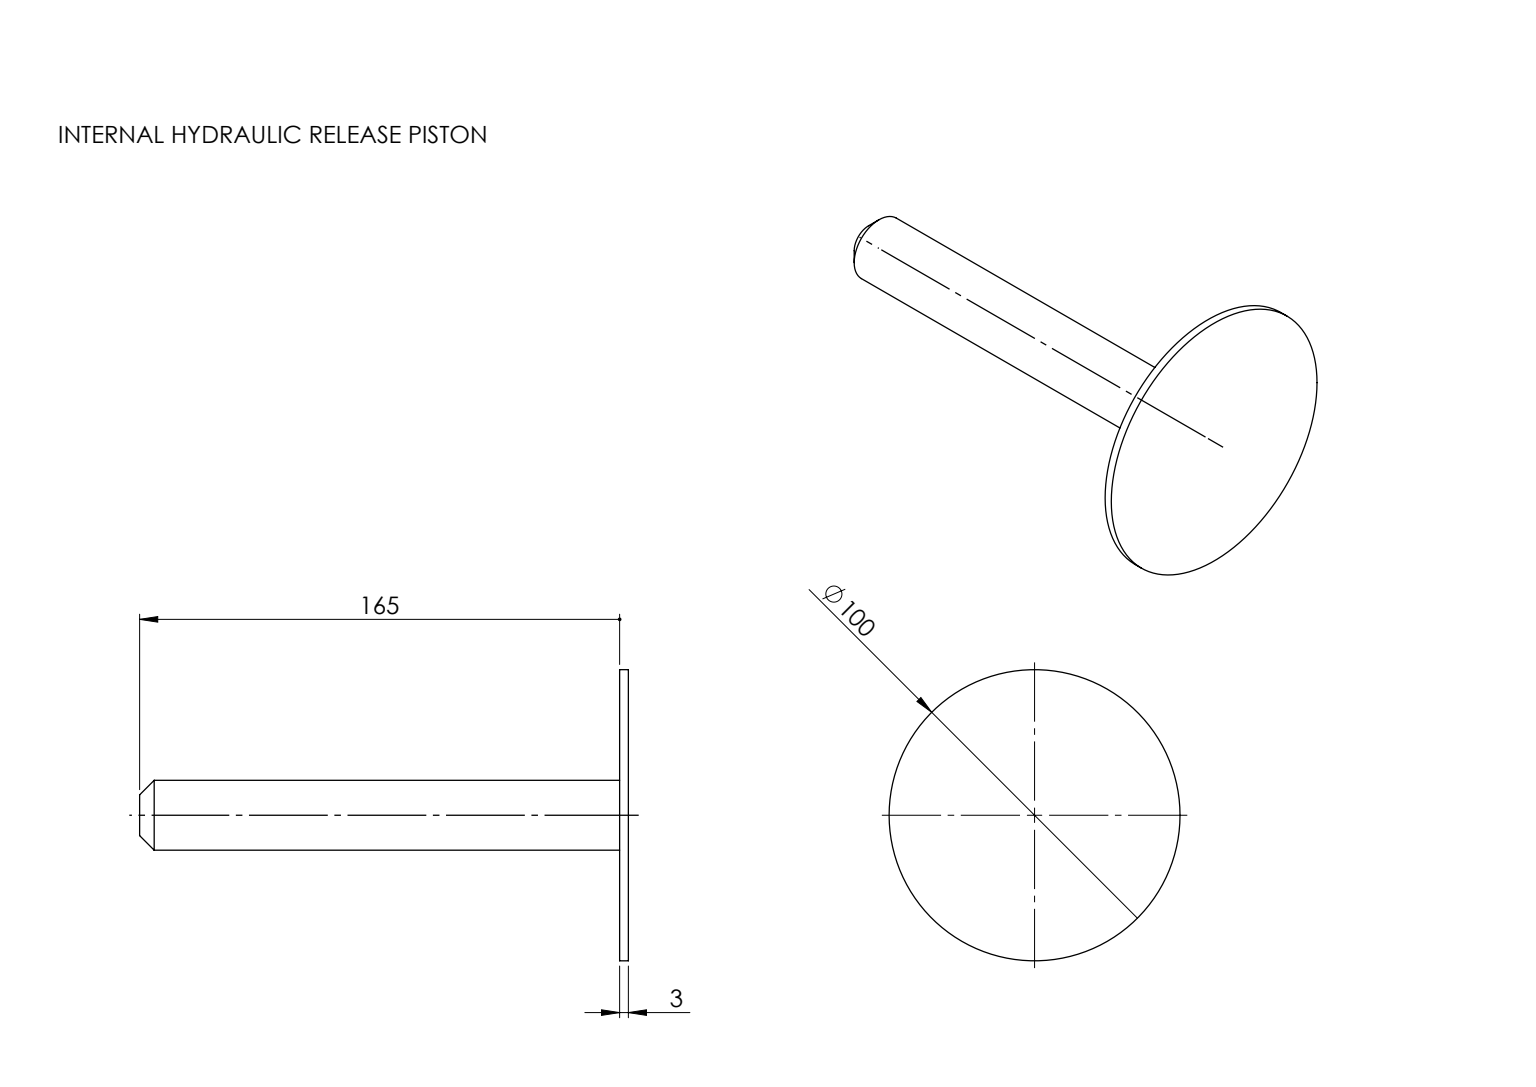
ISO-10303-21;
HEADER;
FILE_DESCRIPTION (('STEP AP214'),
    '1' );
FILE_NAME ('Internal Hydraulic Release Piston.step',
    '2026-10-08T07:58:12',
    ( '' ),
    ( '' ),
    'SwSTEP 2.0',
    'SolidWorks 2026',
    '' );
FILE_SCHEMA (( 'AUTOMOTIVE_DESIGN' ));
ENDSEC;

DATA;
#3=CARTESIAN_POINT ( 'NONE',  ( 112.4999999999999858, 155.0000000000000000, -6.938893903907228378E-15 ) ) ;
#34=EDGE_LOOP ( 'NONE', ( #21556, #29225, #7331, #33094 ) ) ;
#120=ORIENTED_EDGE ( 'NONE', *, *, #31535, .T. ) ;
#168=FILL_AREA_STYLE ('',( #5443 ) ) ;
#368=VECTOR ( 'NONE', #30488, 1000.000000000000000 ) ;
#375=MECHANICAL_DESIGN_GEOMETRIC_PRESENTATION_REPRESENTATION('',(#3643),#27015);
#385=DIRECTION ( 'NONE',  ( -1.000000000000000000, -0.000000000000000000, -0.000000000000000000 ) ) ;
#394=VECTOR ( 'NONE', #33049, 1000.000000000000114 ) ;
#409=EDGE_LOOP ( 'NONE', ( #12808, #6354, #120, #4248 ) ) ;
#672=MANIFOLD_SOLID_BREP ( 'Boss-Extrude2', #22647 ) ;
#768=ORIENTED_EDGE ( 'NONE', *, *, #31535, .F. ) ;
#874=DIRECTION ( 'NONE',  ( 1.000000000000000000, 0.000000000000000000, 0.000000000000000000 ) ) ;
#999=DIRECTION ( 'NONE',  ( 0.000000000000000000, 0.000000000000000000, 1.000000000000000000 ) ) ;
#1205=PRESENTATION_STYLE_ASSIGNMENT (( #14154 ) ) ;
#1257=PRODUCT ( 'Internal Hydraulic Release Piston', 'Internal Hydraulic Release Piston', '', ( #26899 ) ) ;
#1290=AXIS2_PLACEMENT_3D ( 'NONE', #17289, #33134, #30578 ) ;
#1337=VERTEX_POINT ( 'NONE', #24281 ) ;
#1508=AXIS2_PLACEMENT_3D ( 'NONE', #25293, #33136, #15242 ) ;
#1607=EDGE_CURVE ( 'NONE', #8578, #22189, #6963, .T. ) ;
#1664=VERTEX_POINT ( 'NONE', #18314 ) ;
#1670=EDGE_CURVE ( 'NONE', #22189, #8578, #14617, .T. ) ;
#1776=EDGE_LOOP ( 'NONE', ( #1876, #22480, #11969, #27098 ) ) ;
#1840=CYLINDRICAL_SURFACE ( 'NONE', #11781, 12.00000000000000355 ) ;
#1876=ORIENTED_EDGE ( 'NONE', *, *, #16847, .F. ) ;
#1924=ORIENTED_EDGE ( 'NONE', *, *, #23365, .F. ) ;
#2147=CARTESIAN_POINT ( 'NONE',  ( 112.4999999999999858, 155.0000000000000000, -6.938893903907228378E-15 ) ) ;
#2185=SHAPE_REPRESENTATION ( 'Internal Hydraulic Release Piston', ( #2404 ), #27952 ) ;
#2223=DIRECTION ( 'NONE',  ( -1.000000000000000000, -0.000000000000000000, -0.000000000000000000 ) ) ;
#2250=DIRECTION ( 'NONE',  ( 0.000000000000000000, 0.000000000000000000, -1.000000000000000000 ) ) ;
#2404=AXIS2_PLACEMENT_3D ( 'NONE', #8872, #11941, #4266 ) ;
#2565=SHAPE_REPRESENTATION_RELATIONSHIP ( 'NONE' , 'NONE' ,  #2185, #14909 ) ;
#2939=COLOUR_RGB ( '', 0.66274510, 0.83137255, 0.94901961) ;
#3015=FACE_OUTER_BOUND ( 'NONE', #1776, .T. ) ;
#3175=DIRECTION ( 'NONE',  ( -1.000000000000000000, -0.000000000000000000, -0.000000000000000000 ) ) ;
#3218=CARTESIAN_POINT ( 'NONE',  ( 115.4999999999999858, 155.0000000000000000, -6.938893903907228378E-15 ) ) ;
#3386=SHAPE_DEFINITION_REPRESENTATION ( #33668, #2185 ) ;
#3476=( GEOMETRIC_REPRESENTATION_CONTEXT ( 3 ) GLOBAL_UNCERTAINTY_ASSIGNED_CONTEXT ( ( #16111 ) ) GLOBAL_UNIT_ASSIGNED_CONTEXT ( ( #32711, #27439, #10407 ) ) REPRESENTATION_CONTEXT ( 'NONE', 'WORKASPACE' ) );
#3643=STYLED_ITEM ( 'NONE', ( #24499 ), #672 ) ;
#3732=DIRECTION ( 'NONE',  ( 1.000000000000000000, 0.000000000000000000, 0.000000000000000000 ) ) ;
#3769=FILL_AREA_STYLE ('',( #27108 ) ) ;
#4018=MECHANICAL_DESIGN_GEOMETRIC_PRESENTATION_REPRESENTATION('',(#13819),#3476);
#4163=EDGE_CURVE ( 'NONE', #8578, #31129, #13331, .T. ) ;
#4176=CARTESIAN_POINT ( 'NONE',  ( 112.4999999999999858, 155.0000000000000000, -6.938893903907228378E-15 ) ) ;
#4218=DIRECTION ( 'NONE',  ( 0.000000000000000000, 0.000000000000000000, 1.000000000000000000 ) ) ;
#4248=ORIENTED_EDGE ( 'NONE', *, *, #25720, .T. ) ;
#4266=DIRECTION ( 'NONE',  ( 1.000000000000000000, 0.000000000000000000, 0.000000000000000000 ) ) ;
#4522=DIRECTION ( 'NONE',  ( 0.000000000000000000, 0.000000000000000000, -1.000000000000000000 ) ) ;
#4904=LINE ( 'NONE', #22961, #7980 ) ;
#5202=EDGE_CURVE ( 'NONE', #1337, #29025, #8726, .T. ) ;
#5443=FILL_AREA_STYLE_COLOUR ( '', #24313 ) ;
#5628=AXIS2_PLACEMENT_3D ( 'NONE', #4176, #19521, #4522 ) ;
#5888=UNCERTAINTY_MEASURE_WITH_UNIT (LENGTH_MEASURE( 1.000000000000000082E-05 ), #26387, 'distance_accuracy_value', 'NONE');
#6054=VECTOR ( 'NONE', #385, 1000.000000000000000 ) ;
#6112=AXIS2_PLACEMENT_3D ( 'NONE', #22939, #14935, #9482 ) ;
#6312=( NAMED_UNIT ( * ) PLANE_ANGLE_UNIT ( ) SI_UNIT ( $, .RADIAN. ) );
#6354=ORIENTED_EDGE ( 'NONE', *, *, #1670, .F. ) ;
#6598=EDGE_LOOP ( 'NONE', ( #10063, #33597, #18191, #768 ) ) ;
#6737=AXIS2_PLACEMENT_3D ( 'NONE', #20804, #7872, #20130 ) ;
#6963=CIRCLE ( 'NONE', #26011, 12.00000000000000355 ) ;
#7331=ORIENTED_EDGE ( 'NONE', *, *, #29781, .T. ) ;
#7508=CIRCLE ( 'NONE', #1508, 50.00000000000000000 ) ;
#7830=LINE ( 'NONE', #33213, #368 ) ;
#7872=DIRECTION ( 'NONE',  ( 1.000000000000000000, -0.000000000000000000, -0.000000000000000000 ) ) ;
#7939=DIRECTION ( 'NONE',  ( 0.000000000000000000, 0.000000000000000000, -1.000000000000000000 ) ) ;
#7980=VECTOR ( 'NONE', #22285, 1000.000000000000000 ) ;
#7987=CARTESIAN_POINT ( 'NONE',  ( 112.4999999999999858, 155.0000000000000000, -50.00000000000000711 ) ) ;
#8143=CARTESIAN_POINT ( 'NONE',  ( -47.49999999999998579, 155.0000000000000000, -6.938893903907228378E-15 ) ) ;
#8320=CIRCLE ( 'NONE', #6112, 6.999999999999950262 ) ;
#8578=VERTEX_POINT ( 'NONE', #16343 ) ;
#8726=CIRCLE ( 'NONE', #9827, 50.00000000000000000 ) ;
#8740=PRODUCT_DEFINITION_CONTEXT ( 'detailed design', #14200, 'design' ) ;
#8872=CARTESIAN_POINT ( 'NONE',  ( 0.000000000000000000, 0.000000000000000000, 0.000000000000000000 ) ) ;
#8976=APPLICATION_CONTEXT ( 'automotive_design' ) ;
#8992=CARTESIAN_POINT ( 'NONE',  ( -47.49999999999998579, 155.0000000000000000, -6.938893903907228378E-15 ) ) ;
#9056=EDGE_LOOP ( 'NONE', ( #32117, #30050 ) ) ;
#9124=FACE_OUTER_BOUND ( 'NONE', #9056, .T. ) ;
#9187=CARTESIAN_POINT ( 'NONE',  ( 115.4999999999999858, 155.0000000000000000, 49.99999999999999289 ) ) ;
#9216=LINE ( 'NONE', #17385, #394 ) ;
#9316=EDGE_LOOP ( 'NONE', ( #18007, #24239 ) ) ;
#9482=DIRECTION ( 'NONE',  ( 0.000000000000000000, 0.000000000000000000, -1.000000000000000000 ) ) ;
#9529=EDGE_CURVE ( 'NONE', #29025, #1337, #17264, .T. ) ;
#9577=EDGE_CURVE ( 'NONE', #12511, #17462, #9216, .T. ) ;
#9827=AXIS2_PLACEMENT_3D ( 'NONE', #11231, #3732, #24515 ) ;
#9834=EDGE_CURVE ( 'NONE', #1337, #29281, #13277, .T. ) ;
#9984=DIRECTION ( 'NONE',  ( 0.000000000000000000, 0.000000000000000000, -1.000000000000000000 ) ) ;
#9985=AXIS2_PLACEMENT_3D ( 'NONE', #30374, #14691, #22702 ) ;
#10063=ORIENTED_EDGE ( 'NONE', *, *, #1607, .F. ) ;
#10190=ADVANCED_FACE ( 'NONE', ( #11396 ), #24328, .T. ) ;
#10407=( NAMED_UNIT ( * ) SI_UNIT ( $, .STERADIAN. ) SOLID_ANGLE_UNIT ( ) );
#11231=CARTESIAN_POINT ( 'NONE',  ( 115.4999999999999858, 155.0000000000000000, -6.938893903907228378E-15 ) ) ;
#11339=AXIS2_PLACEMENT_3D ( 'NONE', #8992, #21933, #20057 ) ;
#11343=FACE_OUTER_BOUND ( 'NONE', #28185, .T. ) ;
#11392=( NAMED_UNIT ( * ) SI_UNIT ( $, .STERADIAN. ) SOLID_ANGLE_UNIT ( ) );
#11396=FACE_OUTER_BOUND ( 'NONE', #23916, .T. ) ;
#11630=CIRCLE ( 'NONE', #6737, 12.00000000000000355 ) ;
#11774=CARTESIAN_POINT ( 'NONE',  ( -52.50000000000002132, 155.0000000000000000, 6.999999999999944045 ) ) ;
#11781=AXIS2_PLACEMENT_3D ( 'NONE', #25343, #20068, #4218 ) ;
#11844=PLANE ( 'NONE',  #17296 ) ;
#11849=AXIS2_PLACEMENT_3D ( 'NONE', #3, #30839, #22826 ) ;
#11941=DIRECTION ( 'NONE',  ( 0.000000000000000000, 0.000000000000000000, 1.000000000000000000 ) ) ;
#11969=ORIENTED_EDGE ( 'NONE', *, *, #16455, .F. ) ;
#12006=CARTESIAN_POINT ( 'NONE',  ( -52.50000000000002132, 155.0000000000000000, -6.999999999999957367 ) ) ;
#12259=ORIENTED_EDGE ( 'NONE', *, *, #16847, .T. ) ;
#12511=VERTEX_POINT ( 'NONE', #11774 ) ;
#12659=CARTESIAN_POINT ( 'NONE',  ( 112.4999999999999858, 155.0000000000000000, -12.00000000000001066 ) ) ;
#12808=ORIENTED_EDGE ( 'NONE', *, *, #4163, .F. ) ;
#12881=CONICAL_SURFACE ( 'NONE', #17227, 12.00000000000000355, 0.7853981633974503884 ) ;
#12987=VECTOR ( 'NONE', #20204, 1000.000000000000114 ) ;
#13277=LINE ( 'NONE', #23669, #16159 ) ;
#13331=LINE ( 'NONE', #12659, #6054 ) ;
#13384=ORIENTED_EDGE ( 'NONE', *, *, #1670, .T. ) ;
#13499=CIRCLE ( 'NONE', #11339, 12.00000000000000355 ) ;
#13513=ORIENTED_EDGE ( 'NONE', *, *, #22668, .T. ) ;
#13566=CARTESIAN_POINT ( 'NONE',  ( 115.4999999999999858, 155.0000000000000000, -6.938893903907228378E-15 ) ) ;
#13604=DIRECTION ( 'NONE',  ( -1.000000000000000000, -0.000000000000000000, -0.000000000000000000 ) ) ;
#13768=SURFACE_STYLE_USAGE ( .BOTH. , #26218 ) ;
#13818=CARTESIAN_POINT ( 'NONE',  ( 115.4999999999999858, 155.0000000000000000, -6.938893903907228378E-15 ) ) ;
#13819=STYLED_ITEM ( 'NONE', ( #1205 ), #14909 ) ;
#14104=( NAMED_UNIT ( * ) PLANE_ANGLE_UNIT ( ) SI_UNIT ( $, .RADIAN. ) );
#14154=SURFACE_STYLE_USAGE ( .BOTH. , #17044 ) ;
#14200=APPLICATION_CONTEXT ( 'automotive_design' ) ;
#14324=( NAMED_UNIT ( * ) SI_UNIT ( $, .STERADIAN. ) SOLID_ANGLE_UNIT ( ) );
#14470=ORIENTED_EDGE ( 'NONE', *, *, #9834, .T. ) ;
#14617=CIRCLE ( 'NONE', #30955, 12.00000000000000355 ) ;
#14691=DIRECTION ( 'NONE',  ( 1.000000000000000000, -0.000000000000000000, -0.000000000000000000 ) ) ;
#14909=ADVANCED_BREP_SHAPE_REPRESENTATION ( '', ( #672, #2404 ), #27952 ) ;
#14935=DIRECTION ( 'NONE',  ( -1.000000000000000000, -0.000000000000000000, -0.000000000000000000 ) ) ;
#15078=CARTESIAN_POINT ( 'NONE',  ( 112.4999999999999858, 155.0000000000000000, -6.938893903907228378E-15 ) ) ;
#15204=EDGE_CURVE ( 'NONE', #1664, #29281, #27346, .T. ) ;
#15242=DIRECTION ( 'NONE',  ( 0.000000000000000000, 0.000000000000000000, -1.000000000000000000 ) ) ;
#15269=CARTESIAN_POINT ( 'NONE',  ( 112.4999999999999858, 155.0000000000000000, 11.99999999999999645 ) ) ;
#16110=DIRECTION ( 'NONE',  ( 0.000000000000000000, 0.000000000000000000, 1.000000000000000000 ) ) ;
#16111=UNCERTAINTY_MEASURE_WITH_UNIT (LENGTH_MEASURE( 1.000000000000000082E-05 ), #32711, 'distance_accuracy_value', 'NONE');
#16118=DIRECTION ( 'NONE',  ( 1.000000000000000000, -0.000000000000000000, -0.000000000000000000 ) ) ;
#16159=VECTOR ( 'NONE', #2223, 1000.000000000000000 ) ;
#16343=CARTESIAN_POINT ( 'NONE',  ( 112.4999999999999858, 155.0000000000000000, -12.00000000000001066 ) ) ;
#16455=EDGE_CURVE ( 'NONE', #31129, #17462, #11630, .T. ) ;
#16729=DIRECTION ( 'NONE',  ( -1.000000000000000000, -0.000000000000000000, -0.000000000000000000 ) ) ;
#16847=EDGE_CURVE ( 'NONE', #12511, #18640, #8320, .T. ) ;
#17044=SURFACE_SIDE_STYLE ('',( #32377 ) ) ;
#17125=DIRECTION ( 'NONE',  ( 0.000000000000000000, 0.000000000000000000, -1.000000000000000000 ) ) ;
#17227=AXIS2_PLACEMENT_3D ( 'NONE', #8143, #16118, #18195 ) ;
#17264=CIRCLE ( 'NONE', #31919, 50.00000000000000000 ) ;
#17289=CARTESIAN_POINT ( 'NONE',  ( 115.4999999999999858, 155.0000000000000000, -6.938893903907228378E-15 ) ) ;
#17296=AXIS2_PLACEMENT_3D ( 'NONE', #21725, #22232, #17125 ) ;
#17385=CARTESIAN_POINT ( 'NONE',  ( -47.49999999999998579, 155.0000000000000000, 11.99999999999999645 ) ) ;
#17462=VERTEX_POINT ( 'NONE', #22903 ) ;
#17465=FACE_BOUND ( 'NONE', #22519, .T. ) ;
#17627=FACE_OUTER_BOUND ( 'NONE', #9316, .T. ) ;
#18007=ORIENTED_EDGE ( 'NONE', *, *, #9529, .T. ) ;
#18191=ORIENTED_EDGE ( 'NONE', *, *, #16455, .T. ) ;
#18195=DIRECTION ( 'NONE',  ( 0.000000000000000000, 0.000000000000000000, -1.000000000000000000 ) ) ;
#18314=CARTESIAN_POINT ( 'NONE',  ( 112.4999999999999858, 155.0000000000000000, 49.99999999999999289 ) ) ;
#18640=VERTEX_POINT ( 'NONE', #12006 ) ;
#18746=ADVANCED_FACE ( 'NONE', ( #17627 ), #22392, .T. ) ;
#18845=CIRCLE ( 'NONE', #29717, 6.999999999999950262 ) ;
#19521=DIRECTION ( 'NONE',  ( 1.000000000000000000, 0.000000000000000000, 0.000000000000000000 ) ) ;
#19935=( LENGTH_UNIT ( ) NAMED_UNIT ( * ) SI_UNIT ( .MILLI., .METRE. ) );
#20057=DIRECTION ( 'NONE',  ( 0.000000000000000000, 0.000000000000000000, -1.000000000000000000 ) ) ;
#20068=DIRECTION ( 'NONE',  ( -1.000000000000000000, -0.000000000000000000, -0.000000000000000000 ) ) ;
#20130=DIRECTION ( 'NONE',  ( 0.000000000000000000, 0.000000000000000000, -1.000000000000000000 ) ) ;
#20204=DIRECTION ( 'NONE',  ( 0.7071067811865461294, 0.000000000000000000, -0.7071067811865489050 ) ) ;
#20371=DIRECTION ( 'NONE',  ( 1.000000000000000000, 0.000000000000000000, 0.000000000000000000 ) ) ;
#20383=CARTESIAN_POINT ( 'NONE',  ( -47.49999999999998579, 155.0000000000000000, -12.00000000000001066 ) ) ;
#20804=CARTESIAN_POINT ( 'NONE',  ( -47.49999999999998579, 155.0000000000000000, -6.938893903907228378E-15 ) ) ;
#20908=UNCERTAINTY_MEASURE_WITH_UNIT (LENGTH_MEASURE( 1.000000000000000082E-05 ), #19935, 'distance_accuracy_value', 'NONE');
#21045=ADVANCED_FACE ( 'NONE', ( #26506 ), #27304, .T. ) ;
#21221=ORIENTED_EDGE ( 'NONE', *, *, #9834, .F. ) ;
#21375=ADVANCED_FACE ( 'NONE', ( #22356 ), #24658, .T. ) ;
#21556=ORIENTED_EDGE ( 'NONE', *, *, #9577, .F. ) ;
#21652=DIRECTION ( 'NONE',  ( 0.000000000000000000, 0.000000000000000000, -1.000000000000000000 ) ) ;
#21725=CARTESIAN_POINT ( 'NONE',  ( -52.50000000000002132, 155.0000000000000000, -6.938893903907228378E-15 ) ) ;
#21933=DIRECTION ( 'NONE',  ( 1.000000000000000000, -0.000000000000000000, -0.000000000000000000 ) ) ;
#22189=VERTEX_POINT ( 'NONE', #15269 ) ;
#22232=DIRECTION ( 'NONE',  ( 1.000000000000000000, 0.000000000000000000, 0.000000000000000000 ) ) ;
#22285=DIRECTION ( 'NONE',  ( -1.000000000000000000, -0.000000000000000000, -0.000000000000000000 ) ) ;
#22356=FACE_OUTER_BOUND ( 'NONE', #34, .T. ) ;
#22392=PLANE ( 'NONE',  #1290 ) ;
#22456=AXIS2_PLACEMENT_3D ( 'NONE', #25650, #25826, #7939 ) ;
#22480=ORIENTED_EDGE ( 'NONE', *, *, #9577, .T. ) ;
#22519=EDGE_LOOP ( 'NONE', ( #13384, #28528 ) ) ;
#22647=CLOSED_SHELL ( 'NONE', ( #21045, #31754, #25134, #31438, #24360, #21375, #10190, #18746, #33131 ) ) ;
#22668=EDGE_CURVE ( 'NONE', #18640, #12511, #18845, .T. ) ;
#22702=DIRECTION ( 'NONE',  ( 0.000000000000000000, 0.000000000000000000, -1.000000000000000000 ) ) ;
#22786=EDGE_LOOP ( 'NONE', ( #23173, #14470, #28097, #1924 ) ) ;
#22826=DIRECTION ( 'NONE',  ( 0.000000000000000000, 0.000000000000000000, 1.000000000000000000 ) ) ;
#22903=CARTESIAN_POINT ( 'NONE',  ( -47.49999999999998579, 155.0000000000000000, 11.99999999999999645 ) ) ;
#22939=CARTESIAN_POINT ( 'NONE',  ( -52.50000000000002132, 155.0000000000000000, -6.938893903907228378E-15 ) ) ;
#22961=CARTESIAN_POINT ( 'NONE',  ( 112.4999999999999858, 155.0000000000000000, 11.99999999999999645 ) ) ;
#23173=ORIENTED_EDGE ( 'NONE', *, *, #5202, .F. ) ;
#23365=EDGE_CURVE ( 'NONE', #29025, #1664, #7830, .T. ) ;
#23669=CARTESIAN_POINT ( 'NONE',  ( 115.4999999999999858, 155.0000000000000000, -50.00000000000000711 ) ) ;
#23916=EDGE_LOOP ( 'NONE', ( #21221, #24408, #26618, #24605 ) ) ;
#24239=ORIENTED_EDGE ( 'NONE', *, *, #5202, .T. ) ;
#24281=CARTESIAN_POINT ( 'NONE',  ( 115.4999999999999858, 155.0000000000000000, -50.00000000000000711 ) ) ;
#24313=COLOUR_RGB ( '', 0.66274510, 0.83137255, 0.94901961) ;
#24328=CYLINDRICAL_SURFACE ( 'NONE', #28171, 50.00000000000000000 ) ;
#24360=ADVANCED_FACE ( 'NONE', ( #11343 ), #11844, .F. ) ;
#24408=ORIENTED_EDGE ( 'NONE', *, *, #9529, .F. ) ;
#24499=PRESENTATION_STYLE_ASSIGNMENT (( #13768 ) ) ;
#24505=CARTESIAN_POINT ( 'NONE',  ( -47.49999999999998579, 155.0000000000000000, -12.00000000000001066 ) ) ;
#24515=DIRECTION ( 'NONE',  ( 0.000000000000000000, 0.000000000000000000, -1.000000000000000000 ) ) ;
#24542=EDGE_CURVE ( 'NONE', #29281, #1664, #7508, .T. ) ;
#24605=ORIENTED_EDGE ( 'NONE', *, *, #15204, .T. ) ;
#24658=CONICAL_SURFACE ( 'NONE', #9985, 12.00000000000000355, 0.7853981633974503884 ) ;
#25134=ADVANCED_FACE ( 'NONE', ( #25550 ), #31335, .T. ) ;
#25293=CARTESIAN_POINT ( 'NONE',  ( 112.4999999999999858, 155.0000000000000000, -6.938893903907228378E-15 ) ) ;
#25343=CARTESIAN_POINT ( 'NONE',  ( 112.4999999999999858, 155.0000000000000000, -6.938893903907228378E-15 ) ) ;
#25474=DIRECTION ( 'NONE',  ( 1.000000000000000000, 0.000000000000000000, 0.000000000000000000 ) ) ;
#25550=FACE_OUTER_BOUND ( 'NONE', #6598, .T. ) ;
#25650=CARTESIAN_POINT ( 'NONE',  ( 112.4999999999999858, 155.0000000000000000, -6.938893903907228378E-15 ) ) ;
#25719=SURFACE_STYLE_FILL_AREA ( #168 ) ;
#25720=EDGE_CURVE ( 'NONE', #17462, #31129, #13499, .T. ) ;
#25826=DIRECTION ( 'NONE',  ( 1.000000000000000000, 0.000000000000000000, 0.000000000000000000 ) ) ;
#26011=AXIS2_PLACEMENT_3D ( 'NONE', #2147, #20371, #9984 ) ;
#26218=SURFACE_SIDE_STYLE ('',( #25719 ) ) ;
#26387=( LENGTH_UNIT ( ) NAMED_UNIT ( * ) SI_UNIT ( .MILLI., .METRE. ) );
#26506=FACE_OUTER_BOUND ( 'NONE', #22786, .T. ) ;
#26618=ORIENTED_EDGE ( 'NONE', *, *, #23365, .T. ) ;
#26899=PRODUCT_CONTEXT ( 'NONE', #8976, 'mechanical' ) ;
#27015=( GEOMETRIC_REPRESENTATION_CONTEXT ( 3 ) GLOBAL_UNCERTAINTY_ASSIGNED_CONTEXT ( ( #5888 ) ) GLOBAL_UNIT_ASSIGNED_CONTEXT ( ( #26387, #14104, #11392 ) ) REPRESENTATION_CONTEXT ( 'NONE', 'WORKASPACE' ) );
#27098=ORIENTED_EDGE ( 'NONE', *, *, #29781, .F. ) ;
#27108=FILL_AREA_STYLE_COLOUR ( '', #2939 ) ;
#27304=CYLINDRICAL_SURFACE ( 'NONE', #32797, 50.00000000000000000 ) ;
#27346=CIRCLE ( 'NONE', #22456, 50.00000000000000000 ) ;
#27439=( NAMED_UNIT ( * ) PLANE_ANGLE_UNIT ( ) SI_UNIT ( $, .RADIAN. ) );
#27850=PLANE ( 'NONE',  #5628 ) ;
#27952=( GEOMETRIC_REPRESENTATION_CONTEXT ( 3 ) GLOBAL_UNCERTAINTY_ASSIGNED_CONTEXT ( ( #20908 ) ) GLOBAL_UNIT_ASSIGNED_CONTEXT ( ( #19935, #6312, #14324 ) ) REPRESENTATION_CONTEXT ( 'NONE', 'WORKASPACE' ) );
#28097=ORIENTED_EDGE ( 'NONE', *, *, #24542, .T. ) ;
#28171=AXIS2_PLACEMENT_3D ( 'NONE', #3218, #13604, #999 ) ;
#28185=EDGE_LOOP ( 'NONE', ( #13513, #12259 ) ) ;
#28205=DIRECTION ( 'NONE',  ( 0.000000000000000000, 0.000000000000000000, -1.000000000000000000 ) ) ;
#28336=PRODUCT_DEFINITION ( 'UNKNOWN', '', #28422, #8740 ) ;
#28422=PRODUCT_DEFINITION_FORMATION_WITH_SPECIFIED_SOURCE ( 'ANY', '', #1257, .NOT_KNOWN. ) ;
#28528=ORIENTED_EDGE ( 'NONE', *, *, #1607, .T. ) ;
#29025=VERTEX_POINT ( 'NONE', #9187 ) ;
#29225=ORIENTED_EDGE ( 'NONE', *, *, #22668, .F. ) ;
#29281=VERTEX_POINT ( 'NONE', #7987 ) ;
#29683=CARTESIAN_POINT ( 'NONE',  ( -52.50000000000002132, 155.0000000000000000, -6.938893903907228378E-15 ) ) ;
#29717=AXIS2_PLACEMENT_3D ( 'NONE', #29683, #16729, #2250 ) ;
#29781=EDGE_CURVE ( 'NONE', #18640, #31129, #33326, .T. ) ;
#30050=ORIENTED_EDGE ( 'NONE', *, *, #24542, .F. ) ;
#30288=FACE_OUTER_BOUND ( 'NONE', #409, .T. ) ;
#30374=CARTESIAN_POINT ( 'NONE',  ( -47.49999999999998579, 155.0000000000000000, -6.938893903907228378E-15 ) ) ;
#30488=DIRECTION ( 'NONE',  ( -1.000000000000000000, -0.000000000000000000, -0.000000000000000000 ) ) ;
#30578=DIRECTION ( 'NONE',  ( 0.000000000000000000, 0.000000000000000000, -1.000000000000000000 ) ) ;
#30839=DIRECTION ( 'NONE',  ( -1.000000000000000000, -0.000000000000000000, -0.000000000000000000 ) ) ;
#30955=AXIS2_PLACEMENT_3D ( 'NONE', #15078, #25474, #28205 ) ;
#31129=VERTEX_POINT ( 'NONE', #24505 ) ;
#31335=CYLINDRICAL_SURFACE ( 'NONE', #11849, 12.00000000000000355 ) ;
#31438=ADVANCED_FACE ( 'NONE', ( #30288 ), #1840, .T. ) ;
#31535=EDGE_CURVE ( 'NONE', #22189, #17462, #4904, .T. ) ;
#31754=ADVANCED_FACE ( 'NONE', ( #3015 ), #12881, .T. ) ;
#31919=AXIS2_PLACEMENT_3D ( 'NONE', #13818, #874, #21652 ) ;
#32117=ORIENTED_EDGE ( 'NONE', *, *, #15204, .F. ) ;
#32377=SURFACE_STYLE_FILL_AREA ( #3769 ) ;
#32711=( LENGTH_UNIT ( ) NAMED_UNIT ( * ) SI_UNIT ( .MILLI., .METRE. ) );
#32797=AXIS2_PLACEMENT_3D ( 'NONE', #13566, #3175, #16110 ) ;
#33049=DIRECTION ( 'NONE',  ( 0.7071067811865461294, 8.659560562354951347E-17, 0.7071067811865489050 ) ) ;
#33094=ORIENTED_EDGE ( 'NONE', *, *, #25720, .F. ) ;
#33131=ADVANCED_FACE ( 'NONE', ( #17465, #9124 ), #27850, .F. ) ;
#33134=DIRECTION ( 'NONE',  ( 1.000000000000000000, 0.000000000000000000, 0.000000000000000000 ) ) ;
#33136=DIRECTION ( 'NONE',  ( 1.000000000000000000, 0.000000000000000000, 0.000000000000000000 ) ) ;
#33213=CARTESIAN_POINT ( 'NONE',  ( 115.4999999999999858, 155.0000000000000000, 49.99999999999999289 ) ) ;
#33326=LINE ( 'NONE', #20383, #12987 ) ;
#33597=ORIENTED_EDGE ( 'NONE', *, *, #4163, .T. ) ;
#33668=PRODUCT_DEFINITION_SHAPE ( 'NONE', 'NONE',  #28336 ) ;
ENDSEC;
END-ISO-10303-21;
